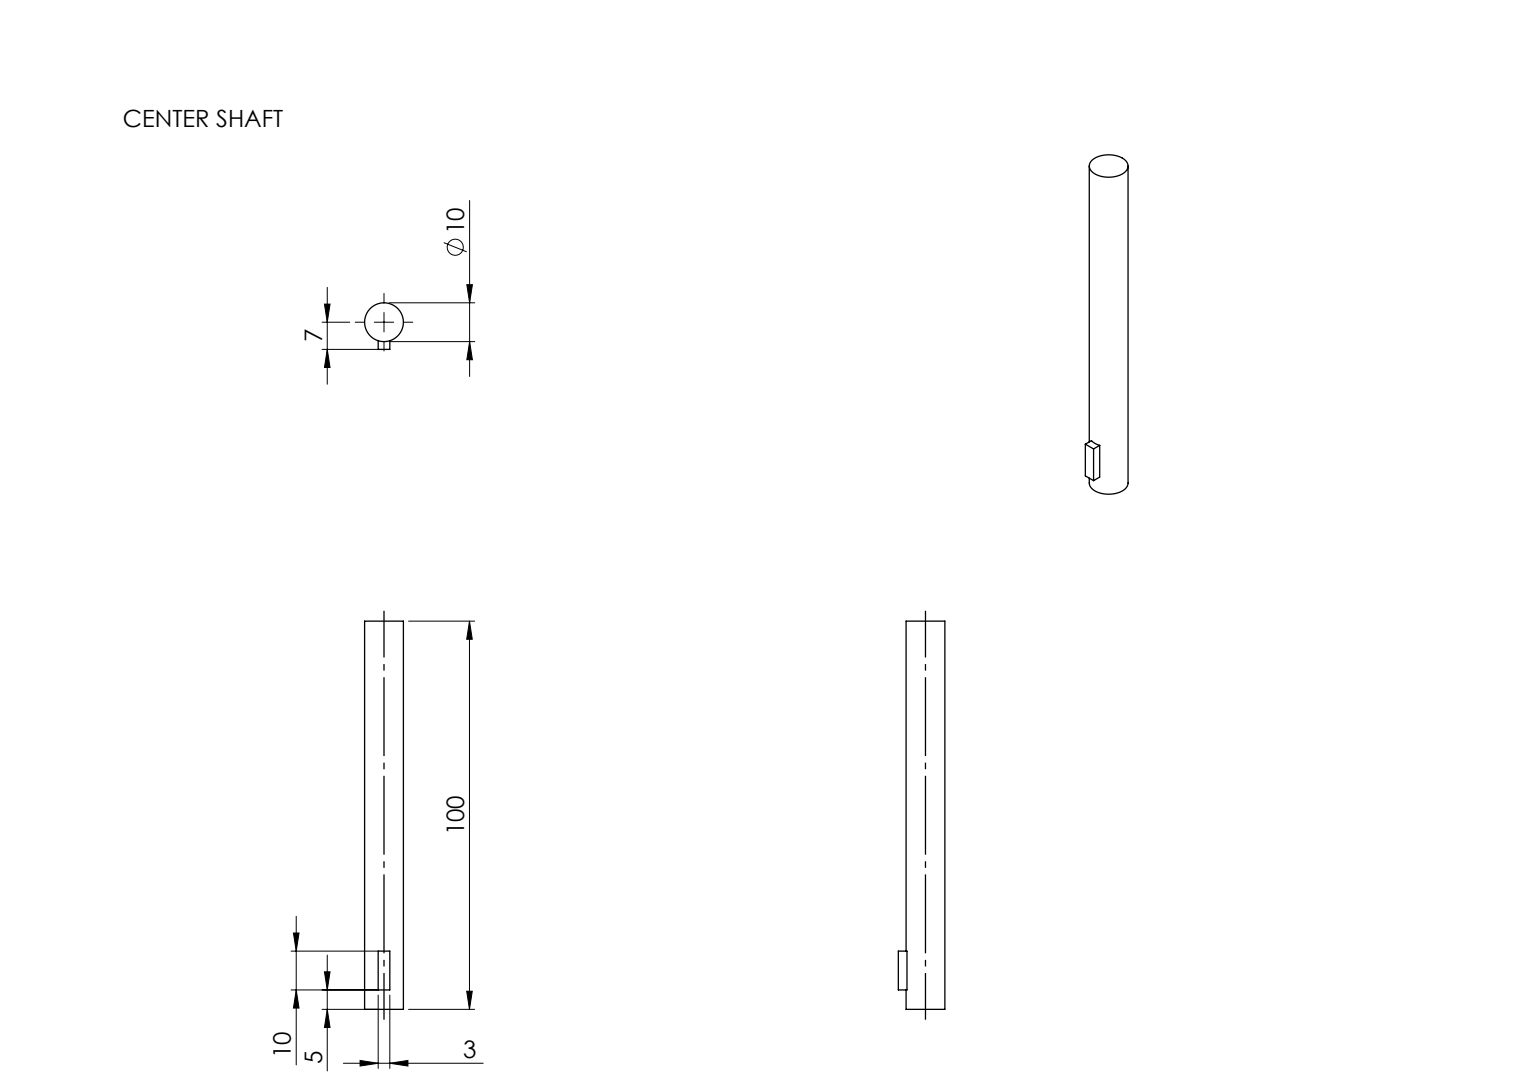
ISO-10303-21;
HEADER;
FILE_DESCRIPTION (('STEP AP214'),
    '1' );
FILE_NAME ('center shaft.step',
    '2026-09-30T13:58:28',
    ( '' ),
    ( '' ),
    'SwSTEP 2.0',
    'SolidWorks 2026',
    '' );
FILE_SCHEMA (( 'AUTOMOTIVE_DESIGN' ));
ENDSEC;

DATA;
#92=CARTESIAN_POINT ( 'NONE',  ( 0.000000000000000000, 100.0000000000000000, 0.000000000000000000 ) ) ;
#95=ADVANCED_FACE ( 'NONE', ( #16404 ), #1281, .F. ) ;
#101=PRODUCT_DEFINITION ( 'UNKNOWN', '', #429, #16859 ) ;
#199=CLOSED_SHELL ( 'NONE', ( #12068, #15575, #17594, #6767, #11084, #7759, #19088, #8385, #95 ) ) ;
#265=EDGE_LOOP ( 'NONE', ( #20128, #1055, #4125, #2694 ) ) ;
#321=EDGE_CURVE ( 'NONE', #616, #3222, #16347, .T. ) ;
#429=PRODUCT_DEFINITION_FORMATION_WITH_SPECIFIED_SOURCE ( 'ANY', '', #11974, .NOT_KNOWN. ) ;
#455=AXIS2_PLACEMENT_3D ( 'NONE', #21743, #16562, #6840 ) ;
#607=DIRECTION ( 'NONE',  ( 0.000000000000000000, 0.000000000000000000, 1.000000000000000000 ) ) ;
#616=VERTEX_POINT ( 'NONE', #12037 ) ;
#674=CARTESIAN_POINT ( 'NONE',  ( 0.000000000000000000, 100.0000000000000000, 0.000000000000000000 ) ) ;
#683=MECHANICAL_DESIGN_GEOMETRIC_PRESENTATION_REPRESENTATION('',(#2802),#19738);
#725=( NAMED_UNIT ( * ) PLANE_ANGLE_UNIT ( ) SI_UNIT ( $, .RADIAN. ) );
#742=EDGE_CURVE ( 'NONE', #12477, #5806, #14229, .T. ) ;
#798=LINE ( 'NONE', #17288, #11093 ) ;
#800=VECTOR ( 'NONE', #14018, 1000.000000000000000 ) ;
#823=FILL_AREA_STYLE_COLOUR ( '', #19105 ) ;
#989=ORIENTED_EDGE ( 'NONE', *, *, #9839, .T. ) ;
#1055=ORIENTED_EDGE ( 'NONE', *, *, #8824, .T. ) ;
#1127=VERTEX_POINT ( 'NONE', #4265 ) ;
#1209=VECTOR ( 'NONE', #5021, 1000.000000000000000 ) ;
#1226=CARTESIAN_POINT ( 'NONE',  ( -1.500000000000000000, 5.000000000000000000, 7.000000000000000000 ) ) ;
#1281=PLANE ( 'NONE',  #4780 ) ;
#1293=DIRECTION ( 'NONE',  ( 0.000000000000000000, -1.000000000000000000, 0.000000000000000000 ) ) ;
#1344=AXIS2_PLACEMENT_3D ( 'NONE', #6692, #13295, #13408 ) ;
#1351=CARTESIAN_POINT ( 'NONE',  ( -1.500000000000000000, 15.00000000000000000, 7.000000000000000000 ) ) ;
#1432=PLANE ( 'NONE',  #13990 ) ;
#1507=ORIENTED_EDGE ( 'NONE', *, *, #15912, .F. ) ;
#1509=ORIENTED_EDGE ( 'NONE', *, *, #20060, .F. ) ;
#1631=APPLICATION_CONTEXT ( 'automotive_design' ) ;
#1753=FACE_OUTER_BOUND ( 'NONE', #3852, .T. ) ;
#1932=ORIENTED_EDGE ( 'NONE', *, *, #19995, .T. ) ;
#1943=( NAMED_UNIT ( * ) PLANE_ANGLE_UNIT ( ) SI_UNIT ( $, .RADIAN. ) );
#2032=DIRECTION ( 'NONE',  ( 0.000000000000000000, 0.000000000000000000, 1.000000000000000000 ) ) ;
#2075=CIRCLE ( 'NONE', #19698, 5.000000000000000000 ) ;
#2102=CARTESIAN_POINT ( 'NONE',  ( 0.000000000000000000, 100.0000000000000000, -5.000000000000000000 ) ) ;
#2151=LINE ( 'NONE', #5477, #19260 ) ;
#2243=DIRECTION ( 'NONE',  ( 0.000000000000000000, 0.000000000000000000, 1.000000000000000000 ) ) ;
#2374=SURFACE_STYLE_USAGE ( .BOTH. , #7253 ) ;
#2502=FACE_OUTER_BOUND ( 'NONE', #20642, .T. ) ;
#2509=ORIENTED_EDGE ( 'NONE', *, *, #11386, .F. ) ;
#2694=ORIENTED_EDGE ( 'NONE', *, *, #321, .F. ) ;
#2772=CARTESIAN_POINT ( 'NONE',  ( -1.500000000000000000, 15.00000000000000000, 0.000000000000000000 ) ) ;
#2791=EDGE_LOOP ( 'NONE', ( #1507, #989, #4089, #3085, #18940 ) ) ;
#2802=STYLED_ITEM ( 'NONE', ( #15197 ), #20649 ) ;
#2947=LINE ( 'NONE', #9672, #7434 ) ;
#2951=CYLINDRICAL_SURFACE ( 'NONE', #10092, 5.000000000000000000 ) ;
#3085=ORIENTED_EDGE ( 'NONE', *, *, #321, .T. ) ;
#3145=FACE_OUTER_BOUND ( 'NONE', #265, .T. ) ;
#3179=CARTESIAN_POINT ( 'NONE',  ( 0.000000000000000000, 100.0000000000000000, 0.000000000000000000 ) ) ;
#3220=PRODUCT_CONTEXT ( 'NONE', #1631, 'mechanical' ) ;
#3222=VERTEX_POINT ( 'NONE', #17271 ) ;
#3230=CARTESIAN_POINT ( 'NONE',  ( 0.000000000000000000, 100.0000000000000000, -5.000000000000000000 ) ) ;
#3247=PLANE ( 'NONE',  #11760 ) ;
#3300=VERTEX_POINT ( 'NONE', #14049 ) ;
#3320=PRODUCT_DEFINITION_SHAPE ( 'NONE', 'NONE',  #101 ) ;
#3361=CARTESIAN_POINT ( 'NONE',  ( 0.000000000000000000, 5.000000000000004441, 0.000000000000000000 ) ) ;
#3443=ORIENTED_EDGE ( 'NONE', *, *, #17842, .T. ) ;
#3468=ORIENTED_EDGE ( 'NONE', *, *, #18425, .F. ) ;
#3530=VERTEX_POINT ( 'NONE', #1226 ) ;
#3670=EDGE_LOOP ( 'NONE', ( #9750, #16754, #6405, #15038, #9979 ) ) ;
#3852=EDGE_LOOP ( 'NONE', ( #3468, #5746 ) ) ;
#3925=( GEOMETRIC_REPRESENTATION_CONTEXT ( 3 ) GLOBAL_UNCERTAINTY_ASSIGNED_CONTEXT ( ( #11439 ) ) GLOBAL_UNIT_ASSIGNED_CONTEXT ( ( #13771, #12002, #13329 ) ) REPRESENTATION_CONTEXT ( 'NONE', 'WORKASPACE' ) );
#4089=ORIENTED_EDGE ( 'NONE', *, *, #13808, .T. ) ;
#4125=ORIENTED_EDGE ( 'NONE', *, *, #12182, .F. ) ;
#4147=( NAMED_UNIT ( * ) SI_UNIT ( $, .STERADIAN. ) SOLID_ANGLE_UNIT ( ) );
#4205=ORIENTED_EDGE ( 'NONE', *, *, #742, .T. ) ;
#4244=CARTESIAN_POINT ( 'NONE',  ( 6.123233995736766282E-16, 100.0000000000000000, 5.000000000000000000 ) ) ;
#4265=CARTESIAN_POINT ( 'NONE',  ( 6.123233995736766282E-16, 0.000000000000000000, 5.000000000000000000 ) ) ;
#4349=EDGE_CURVE ( 'NONE', #20466, #11655, #2075, .T. ) ;
#4384=CARTESIAN_POINT ( 'NONE',  ( -1.500000000000000000, 5.000000000000000000, 7.000000000000000000 ) ) ;
#4780=AXIS2_PLACEMENT_3D ( 'NONE', #19941, #11549, #8018 ) ;
#4823=DIRECTION ( 'NONE',  ( 0.000000000000000000, 0.000000000000000000, -1.000000000000000000 ) ) ;
#4851=VECTOR ( 'NONE', #14439, 1000.000000000000000 ) ;
#4937=COLOUR_RGB ( '', 0.09019608, 0.27058824, 0.51372549) ;
#5017=DIRECTION ( 'NONE',  ( -0.000000000000000000, 0.000000000000000000, -1.000000000000000000 ) ) ;
#5021=DIRECTION ( 'NONE',  ( 0.000000000000000000, -1.000000000000000000, 0.000000000000000000 ) ) ;
#5043=SURFACE_STYLE_USAGE ( .BOTH. , #13323 ) ;
#5212=LINE ( 'NONE', #10500, #21204 ) ;
#5238=CARTESIAN_POINT ( 'NONE',  ( -1.500000000000000000, 5.000000000000004441, 4.769696007084728073 ) ) ;
#5247=LINE ( 'NONE', #15394, #1209 ) ;
#5477=CARTESIAN_POINT ( 'NONE',  ( 1.500000000000000000, 15.00000000000000000, 0.000000000000000000 ) ) ;
#5531=DIRECTION ( 'NONE',  ( 0.000000000000000000, 0.000000000000000000, 1.000000000000000000 ) ) ;
#5556=CARTESIAN_POINT ( 'NONE',  ( 6.123233995736766282E-16, 15.00000000000000000, 5.000000000000000000 ) ) ;
#5679=( GEOMETRIC_REPRESENTATION_CONTEXT ( 3 ) GLOBAL_UNCERTAINTY_ASSIGNED_CONTEXT ( ( #16530 ) ) GLOBAL_UNIT_ASSIGNED_CONTEXT ( ( #15634, #725, #4147 ) ) REPRESENTATION_CONTEXT ( 'NONE', 'WORKASPACE' ) );
#5746=ORIENTED_EDGE ( 'NONE', *, *, #4349, .F. ) ;
#5806=VERTEX_POINT ( 'NONE', #10160 ) ;
#5839=FACE_OUTER_BOUND ( 'NONE', #21460, .T. ) ;
#5917=SHAPE_REPRESENTATION_RELATIONSHIP ( 'NONE' , 'NONE' ,  #21798, #14875 ) ;
#5959=VECTOR ( 'NONE', #11292, 1000.000000000000000 ) ;
#6120=VECTOR ( 'NONE', #9359, 1000.000000000000000 ) ;
#6326=EDGE_CURVE ( 'NONE', #9874, #3300, #9010, .T. ) ;
#6373=EDGE_LOOP ( 'NONE', ( #19171, #4205, #13352, #17793 ) ) ;
#6384=CARTESIAN_POINT ( 'NONE',  ( 1.500000000000000000, 15.00000000000000000, 0.000000000000000000 ) ) ;
#6386=UNCERTAINTY_MEASURE_WITH_UNIT (LENGTH_MEASURE( 1.000000000000000082E-05 ), #11681, 'distance_accuracy_value', 'NONE');
#6403=DIRECTION ( 'NONE',  ( 0.000000000000000000, -1.000000000000000000, 0.000000000000000000 ) ) ;
#6405=ORIENTED_EDGE ( 'NONE', *, *, #17842, .F. ) ;
#6414=STYLED_ITEM ( 'NONE', ( #19070 ), #14875 ) ;
#6551=ORIENTED_EDGE ( 'NONE', *, *, #21621, .T. ) ;
#6596=PLANE ( 'NONE',  #17058 ) ;
#6692=CARTESIAN_POINT ( 'NONE',  ( 0.000000000000000000, 100.0000000000000000, 0.000000000000000000 ) ) ;
#6767=ADVANCED_FACE ( 'NONE', ( #12202 ), #6917, .T. ) ;
#6840=DIRECTION ( 'NONE',  ( 0.000000000000000000, 0.000000000000000000, 1.000000000000000000 ) ) ;
#6917=PLANE ( 'NONE',  #14621 ) ;
#6948=CARTESIAN_POINT ( 'NONE',  ( 1.500000000000000000, 15.00000000000000000, 7.000000000000000000 ) ) ;
#7066=ORIENTED_EDGE ( 'NONE', *, *, #7566, .T. ) ;
#7140=FACE_OUTER_BOUND ( 'NONE', #2791, .T. ) ;
#7253=SURFACE_SIDE_STYLE ('',( #20728 ) ) ;
#7366=FILL_AREA_STYLE ('',( #823 ) ) ;
#7418=DIRECTION ( 'NONE',  ( 0.000000000000000000, -1.000000000000000000, 0.000000000000000000 ) ) ;
#7419=ORIENTED_EDGE ( 'NONE', *, *, #8672, .T. ) ;
#7434=VECTOR ( 'NONE', #18325, 1000.000000000000000 ) ;
#7467=ORIENTED_EDGE ( 'NONE', *, *, #11386, .T. ) ;
#7566=EDGE_CURVE ( 'NONE', #11073, #19781, #13486, .T. ) ;
#7614=DIRECTION ( 'NONE',  ( -0.000000000000000000, -1.000000000000000000, -0.000000000000000000 ) ) ;
#7759=ADVANCED_FACE ( 'NONE', ( #3145 ), #3247, .F. ) ;
#8018=DIRECTION ( 'NONE',  ( -1.000000000000000000, 0.000000000000000000, 0.000000000000000000 ) ) ;
#8056=CIRCLE ( 'NONE', #1344, 5.000000000000000000 ) ;
#8276=DIRECTION ( 'NONE',  ( 0.000000000000000000, -1.000000000000000000, 0.000000000000000000 ) ) ;
#8358=( NAMED_UNIT ( * ) SI_UNIT ( $, .STERADIAN. ) SOLID_ANGLE_UNIT ( ) );
#8385=ADVANCED_FACE ( 'NONE', ( #7140 ), #17414, .T. ) ;
#8462=DIRECTION ( 'NONE',  ( 0.000000000000000000, -0.000000000000000000, -1.000000000000000000 ) ) ;
#8616=CIRCLE ( 'NONE', #15680, 5.000000000000000000 ) ;
#8628=EDGE_CURVE ( 'NONE', #12477, #11073, #19544, .T. ) ;
#8670=CARTESIAN_POINT ( 'NONE',  ( 0.000000000000000000, 0.000000000000000000, 0.000000000000000000 ) ) ;
#8672=EDGE_CURVE ( 'NONE', #11073, #1127, #5247, .T. ) ;
#8824=EDGE_CURVE ( 'NONE', #19781, #3530, #798, .T. ) ;
#9010=LINE ( 'NONE', #6948, #18478 ) ;
#9228=CYLINDRICAL_SURFACE ( 'NONE', #11282, 5.000000000000000000 ) ;
#9258=ORIENTED_EDGE ( 'NONE', *, *, #8628, .T. ) ;
#9359=DIRECTION ( 'NONE',  ( -0.000000000000000000, 1.000000000000000000, -0.000000000000000000 ) ) ;
#9456=PLANE ( 'NONE',  #12316 ) ;
#9564=CARTESIAN_POINT ( 'NONE',  ( -1.500000000000000000, 15.00000000000000000, 7.000000000000000000 ) ) ;
#9591=ORIENTED_EDGE ( 'NONE', *, *, #4349, .T. ) ;
#9672=CARTESIAN_POINT ( 'NONE',  ( -1.500000000000000000, 100.0000000000000000, 4.769696007084728073 ) ) ;
#9750=ORIENTED_EDGE ( 'NONE', *, *, #8628, .F. ) ;
#9839=EDGE_CURVE ( 'NONE', #5806, #18737, #8616, .T. ) ;
#9874=VERTEX_POINT ( 'NONE', #14862 ) ;
#9921=CARTESIAN_POINT ( 'NONE',  ( 0.000000000000000000, 0.000000000000000000, 0.000000000000000000 ) ) ;
#9977=DIRECTION ( 'NONE',  ( 1.000000000000000000, 0.000000000000000000, -0.000000000000000000 ) ) ;
#9979=ORIENTED_EDGE ( 'NONE', *, *, #7566, .F. ) ;
#10092=AXIS2_PLACEMENT_3D ( 'NONE', #3179, #6403, #16434 ) ;
#10097=DIRECTION ( 'NONE',  ( -3.552713678800500929E-15, 0.000000000000000000, 1.000000000000000000 ) ) ;
#10160=CARTESIAN_POINT ( 'NONE',  ( 1.500000000000000000, 15.00000000000000000, 4.769696007084728073 ) ) ;
#10500=CARTESIAN_POINT ( 'NONE',  ( 1.500000000000000000, 5.000000000000000000, 0.000000000000000000 ) ) ;
#10564=DIRECTION ( 'NONE',  ( -1.000000000000000000, 0.000000000000000000, 0.000000000000000000 ) ) ;
#10567=ORIENTED_EDGE ( 'NONE', *, *, #13808, .F. ) ;
#10583=ORIENTED_EDGE ( 'NONE', *, *, #10930, .T. ) ;
#10598=LINE ( 'NONE', #2102, #800 ) ;
#10728=AXIS2_PLACEMENT_3D ( 'NONE', #3361, #15069, #10097 ) ;
#10930=EDGE_CURVE ( 'NONE', #11655, #11594, #10598, .T. ) ;
#11023=DIRECTION ( 'NONE',  ( 1.000000000000000000, 0.000000000000000000, -0.000000000000000000 ) ) ;
#11073=VERTEX_POINT ( 'NONE', #15997 ) ;
#11084=ADVANCED_FACE ( 'NONE', ( #13196 ), #6596, .T. ) ;
#11093=VECTOR ( 'NONE', #2032, 1000.000000000000000 ) ;
#11239=DIRECTION ( 'NONE',  ( -1.000000000000000000, 0.000000000000000000, -0.000000000000000000 ) ) ;
#11254=AXIS2_PLACEMENT_3D ( 'NONE', #9921, #16663, #12789 ) ;
#11282=AXIS2_PLACEMENT_3D ( 'NONE', #18312, #1293, #4823 ) ;
#11292=DIRECTION ( 'NONE',  ( 1.000000000000000000, 0.000000000000000000, 0.000000000000000000 ) ) ;
#11386=EDGE_CURVE ( 'NONE', #20466, #18737, #17396, .T. ) ;
#11439=UNCERTAINTY_MEASURE_WITH_UNIT (LENGTH_MEASURE( 1.000000000000000082E-05 ), #13771, 'distance_accuracy_value', 'NONE');
#11537=AXIS2_PLACEMENT_3D ( 'NONE', #17455, #7614, #19323 ) ;
#11549=DIRECTION ( 'NONE',  ( 0.000000000000000000, 1.000000000000000000, 0.000000000000000000 ) ) ;
#11594=VERTEX_POINT ( 'NONE', #16499 ) ;
#11655=VERTEX_POINT ( 'NONE', #3230 ) ;
#11681=( LENGTH_UNIT ( ) NAMED_UNIT ( * ) SI_UNIT ( .MILLI., .METRE. ) );
#11760=AXIS2_PLACEMENT_3D ( 'NONE', #13301, #9977, #5017 ) ;
#11974=PRODUCT ( 'center shaft', 'center shaft', '', ( #3220 ) ) ;
#12002=( NAMED_UNIT ( * ) PLANE_ANGLE_UNIT ( ) SI_UNIT ( $, .RADIAN. ) );
#12037=CARTESIAN_POINT ( 'NONE',  ( -1.500000000000000000, 15.00000000000000000, 4.769696007084728073 ) ) ;
#12068=ADVANCED_FACE ( 'NONE', ( #17999 ), #2951, .T. ) ;
#12133=AXIS2_PLACEMENT_3D ( 'NONE', #12540, #20617, #10564 ) ;
#12182=EDGE_CURVE ( 'NONE', #3222, #3530, #21295, .T. ) ;
#12202=FACE_OUTER_BOUND ( 'NONE', #16612, .T. ) ;
#12316=AXIS2_PLACEMENT_3D ( 'NONE', #17764, #19307, #11239 ) ;
#12375=ORIENTED_EDGE ( 'NONE', *, *, #12182, .T. ) ;
#12423=VECTOR ( 'NONE', #2243, 1000.000000000000000 ) ;
#12477=VERTEX_POINT ( 'NONE', #20950 ) ;
#12500=DIRECTION ( 'NONE',  ( 0.000000000000000000, 0.000000000000000000, -1.000000000000000000 ) ) ;
#12540=CARTESIAN_POINT ( 'NONE',  ( 0.000000000000000000, 15.00000000000000000, 0.000000000000000000 ) ) ;
#12662=CIRCLE ( 'NONE', #11254, 5.000000000000000000 ) ;
#12789=DIRECTION ( 'NONE',  ( 0.000000000000000000, 0.000000000000000000, -1.000000000000000000 ) ) ;
#12997=CIRCLE ( 'NONE', #21816, 5.000000000000000000 ) ;
#13196=FACE_OUTER_BOUND ( 'NONE', #6373, .T. ) ;
#13295=DIRECTION ( 'NONE',  ( 0.000000000000000000, -1.000000000000000000, 0.000000000000000000 ) ) ;
#13301=CARTESIAN_POINT ( 'NONE',  ( -1.500000000000000000, 15.00000000000000000, 0.000000000000000000 ) ) ;
#13323=SURFACE_SIDE_STYLE ('',( #17081 ) ) ;
#13329=( NAMED_UNIT ( * ) SI_UNIT ( $, .STERADIAN. ) SOLID_ANGLE_UNIT ( ) );
#13352=ORIENTED_EDGE ( 'NONE', *, *, #15912, .T. ) ;
#13408=DIRECTION ( 'NONE',  ( 0.000000000000000000, 0.000000000000000000, -1.000000000000000000 ) ) ;
#13486=CIRCLE ( 'NONE', #455, 5.000000000000000000 ) ;
#13771=( LENGTH_UNIT ( ) NAMED_UNIT ( * ) SI_UNIT ( .MILLI., .METRE. ) );
#13808=EDGE_CURVE ( 'NONE', #18737, #616, #16831, .T. ) ;
#13990=AXIS2_PLACEMENT_3D ( 'NONE', #92, #8276, #16667 ) ;
#14018=DIRECTION ( 'NONE',  ( 0.000000000000000000, -1.000000000000000000, 0.000000000000000000 ) ) ;
#14049=CARTESIAN_POINT ( 'NONE',  ( 1.500000000000000000, 5.000000000000000000, 7.000000000000000000 ) ) ;
#14229=LINE ( 'NONE', #15993, #6120 ) ;
#14439=DIRECTION ( 'NONE',  ( 1.000000000000000000, 0.000000000000000000, 0.000000000000000000 ) ) ;
#14533=CARTESIAN_POINT ( 'NONE',  ( 0.000000000000000000, 15.00000000000000000, 0.000000000000000000 ) ) ;
#14553=DIRECTION ( 'NONE',  ( 0.000000000000000000, -1.000000000000000000, 0.000000000000000000 ) ) ;
#14621=AXIS2_PLACEMENT_3D ( 'NONE', #8670, #18839, #8462 ) ;
#14776=ORIENTED_EDGE ( 'NONE', *, *, #15183, .T. ) ;
#14862=CARTESIAN_POINT ( 'NONE',  ( 1.500000000000000000, 15.00000000000000000, 7.000000000000000000 ) ) ;
#14875=ADVANCED_BREP_SHAPE_REPRESENTATION ( '', ( #20649, #15567 ), #3925 ) ;
#14971=ORIENTED_EDGE ( 'NONE', *, *, #742, .F. ) ;
#15038=ORIENTED_EDGE ( 'NONE', *, *, #8824, .F. ) ;
#15045=SHAPE_DEFINITION_REPRESENTATION ( #3320, #21798 ) ;
#15069=DIRECTION ( 'NONE',  ( -0.000000000000000000, -1.000000000000000000, -0.000000000000000000 ) ) ;
#15183=EDGE_CURVE ( 'NONE', #1127, #11594, #12662, .T. ) ;
#15197=PRESENTATION_STYLE_ASSIGNMENT (( #5043 ) ) ;
#15394=CARTESIAN_POINT ( 'NONE',  ( 6.123233995736766282E-16, 100.0000000000000000, 5.000000000000000000 ) ) ;
#15434=DIRECTION ( 'NONE',  ( 0.000000000000000000, -1.000000000000000000, 0.000000000000000000 ) ) ;
#15567=AXIS2_PLACEMENT_3D ( 'NONE', #21837, #20187, #17085 ) ;
#15575=ADVANCED_FACE ( 'NONE', ( #2502 ), #9228, .T. ) ;
#15634=( LENGTH_UNIT ( ) NAMED_UNIT ( * ) SI_UNIT ( .MILLI., .METRE. ) );
#15680=AXIS2_PLACEMENT_3D ( 'NONE', #14533, #19944, #21275 ) ;
#15886=CARTESIAN_POINT ( 'NONE',  ( 6.123233995736766282E-16, 100.0000000000000000, 5.000000000000000000 ) ) ;
#15912=EDGE_CURVE ( 'NONE', #5806, #9874, #2151, .T. ) ;
#15993=CARTESIAN_POINT ( 'NONE',  ( 1.500000000000000000, 100.0000000000000000, 4.769696007084728073 ) ) ;
#15997=CARTESIAN_POINT ( 'NONE',  ( 6.123233995736766282E-16, 5.000000000000004441, 5.000000000000000000 ) ) ;
#16347=LINE ( 'NONE', #2772, #12423 ) ;
#16404=FACE_OUTER_BOUND ( 'NONE', #3670, .T. ) ;
#16434=DIRECTION ( 'NONE',  ( 0.000000000000000000, 0.000000000000000000, -1.000000000000000000 ) ) ;
#16499=CARTESIAN_POINT ( 'NONE',  ( 0.000000000000000000, 0.000000000000000000, -5.000000000000000000 ) ) ;
#16530=UNCERTAINTY_MEASURE_WITH_UNIT (LENGTH_MEASURE( 1.000000000000000082E-05 ), #15634, 'distance_accuracy_value', 'NONE');
#16562=DIRECTION ( 'NONE',  ( -0.000000000000000000, -1.000000000000000000, -0.000000000000000000 ) ) ;
#16572=ORIENTED_EDGE ( 'NONE', *, *, #8672, .F. ) ;
#16612=EDGE_LOOP ( 'NONE', ( #1932, #14776 ) ) ;
#16636=DIRECTION ( 'NONE',  ( -0.000000000000000000, 0.000000000000000000, -1.000000000000000000 ) ) ;
#16663=DIRECTION ( 'NONE',  ( 0.000000000000000000, -1.000000000000000000, 0.000000000000000000 ) ) ;
#16667=DIRECTION ( 'NONE',  ( 0.000000000000000000, -0.000000000000000000, -1.000000000000000000 ) ) ;
#16673=ORIENTED_EDGE ( 'NONE', *, *, #10930, .F. ) ;
#16754=ORIENTED_EDGE ( 'NONE', *, *, #21484, .T. ) ;
#16831=CIRCLE ( 'NONE', #11537, 5.000000000000000000 ) ;
#16859=PRODUCT_DEFINITION_CONTEXT ( 'detailed design', #19692, 'design' ) ;
#16956=ORIENTED_EDGE ( 'NONE', *, *, #19995, .F. ) ;
#17032=DIRECTION ( 'NONE',  ( 0.000000000000000000, 0.000000000000000000, -1.000000000000000000 ) ) ;
#17058=AXIS2_PLACEMENT_3D ( 'NONE', #6384, #11023, #16636 ) ;
#17081=SURFACE_STYLE_FILL_AREA ( #20080 ) ;
#17085=DIRECTION ( 'NONE',  ( 1.000000000000000000, 0.000000000000000000, 0.000000000000000000 ) ) ;
#17271=CARTESIAN_POINT ( 'NONE',  ( -1.500000000000000000, 15.00000000000000000, 7.000000000000000000 ) ) ;
#17288=CARTESIAN_POINT ( 'NONE',  ( -1.500000000000000000, 5.000000000000000000, 0.000000000000000000 ) ) ;
#17396=LINE ( 'NONE', #4244, #21310 ) ;
#17414=PLANE ( 'NONE',  #12133 ) ;
#17455=CARTESIAN_POINT ( 'NONE',  ( 0.000000000000000000, 15.00000000000000000, 0.000000000000000000 ) ) ;
#17594=ADVANCED_FACE ( 'NONE', ( #1753 ), #1432, .F. ) ;
#17684=MECHANICAL_DESIGN_GEOMETRIC_PRESENTATION_REPRESENTATION('',(#6414),#5679);
#17742=ORIENTED_EDGE ( 'NONE', *, *, #18425, .T. ) ;
#17764=CARTESIAN_POINT ( 'NONE',  ( -1.500000000000000000, 15.00000000000000000, 7.000000000000000000 ) ) ;
#17793=ORIENTED_EDGE ( 'NONE', *, *, #6326, .T. ) ;
#17833=DIRECTION ( 'NONE',  ( 0.000000000000000000, -1.000000000000000000, 0.000000000000000000 ) ) ;
#17842=EDGE_CURVE ( 'NONE', #3530, #3300, #17875, .T. ) ;
#17875=LINE ( 'NONE', #4384, #4851 ) ;
#17999=FACE_OUTER_BOUND ( 'NONE', #18572, .T. ) ;
#18233=ORIENTED_EDGE ( 'NONE', *, *, #6326, .F. ) ;
#18312=CARTESIAN_POINT ( 'NONE',  ( 0.000000000000000000, 100.0000000000000000, 0.000000000000000000 ) ) ;
#18325=DIRECTION ( 'NONE',  ( -0.000000000000000000, 1.000000000000000000, -0.000000000000000000 ) ) ;
#18425=EDGE_CURVE ( 'NONE', #11655, #20466, #8056, .T. ) ;
#18478=VECTOR ( 'NONE', #15434, 1000.000000000000000 ) ;
#18531=VECTOR ( 'NONE', #14553, 1000.000000000000000 ) ;
#18572=EDGE_LOOP ( 'NONE', ( #17742, #7467, #19840, #14971, #9258, #7419, #16956, #16673 ) ) ;
#18737=VERTEX_POINT ( 'NONE', #5556 ) ;
#18839=DIRECTION ( 'NONE',  ( 0.000000000000000000, -1.000000000000000000, 0.000000000000000000 ) ) ;
#18940=ORIENTED_EDGE ( 'NONE', *, *, #20060, .T. ) ;
#19070=PRESENTATION_STYLE_ASSIGNMENT (( #2374 ) ) ;
#19088=ADVANCED_FACE ( 'NONE', ( #5839 ), #9456, .F. ) ;
#19105=COLOUR_RGB ( '', 0.09019608, 0.27058824, 0.51372549) ;
#19171=ORIENTED_EDGE ( 'NONE', *, *, #21484, .F. ) ;
#19260=VECTOR ( 'NONE', #607, 1000.000000000000000 ) ;
#19307=DIRECTION ( 'NONE',  ( 0.000000000000000000, 0.000000000000000000, -1.000000000000000000 ) ) ;
#19323=DIRECTION ( 'NONE',  ( 0.000000000000000000, 0.000000000000000000, 1.000000000000000000 ) ) ;
#19465=CARTESIAN_POINT ( 'NONE',  ( 0.000000000000000000, 0.000000000000000000, 0.000000000000000000 ) ) ;
#19544=CIRCLE ( 'NONE', #10728, 5.000000000000000000 ) ;
#19692=APPLICATION_CONTEXT ( 'automotive_design' ) ;
#19698=AXIS2_PLACEMENT_3D ( 'NONE', #674, #7418, #17032 ) ;
#19738=( GEOMETRIC_REPRESENTATION_CONTEXT ( 3 ) GLOBAL_UNCERTAINTY_ASSIGNED_CONTEXT ( ( #6386 ) ) GLOBAL_UNIT_ASSIGNED_CONTEXT ( ( #11681, #1943, #8358 ) ) REPRESENTATION_CONTEXT ( 'NONE', 'WORKASPACE' ) );
#19781=VERTEX_POINT ( 'NONE', #5238 ) ;
#19799=LINE ( 'NONE', #1351, #5959 ) ;
#19840=ORIENTED_EDGE ( 'NONE', *, *, #9839, .F. ) ;
#19941=CARTESIAN_POINT ( 'NONE',  ( 0.000000000000000000, 5.000000000000000000, 0.000000000000000000 ) ) ;
#19944=DIRECTION ( 'NONE',  ( -0.000000000000000000, -1.000000000000000000, -0.000000000000000000 ) ) ;
#19995=EDGE_CURVE ( 'NONE', #11594, #1127, #12997, .T. ) ;
#20060=EDGE_CURVE ( 'NONE', #3222, #9874, #19799, .T. ) ;
#20080=FILL_AREA_STYLE ('',( #21724 ) ) ;
#20128=ORIENTED_EDGE ( 'NONE', *, *, #21621, .F. ) ;
#20187=DIRECTION ( 'NONE',  ( 0.000000000000000000, 0.000000000000000000, 1.000000000000000000 ) ) ;
#20466=VERTEX_POINT ( 'NONE', #15886 ) ;
#20556=ORIENTED_EDGE ( 'NONE', *, *, #15183, .F. ) ;
#20617=DIRECTION ( 'NONE',  ( 0.000000000000000000, 1.000000000000000000, 0.000000000000000000 ) ) ;
#20642=EDGE_LOOP ( 'NONE', ( #2509, #9591, #10583, #20556, #16572, #7066, #6551, #10567 ) ) ;
#20649=MANIFOLD_SOLID_BREP ( 'Extrude-Thin1', #199 ) ;
#20728=SURFACE_STYLE_FILL_AREA ( #7366 ) ;
#20905=DIRECTION ( 'NONE',  ( 0.000000000000000000, -1.000000000000000000, 0.000000000000000000 ) ) ;
#20950=CARTESIAN_POINT ( 'NONE',  ( 1.500000000000000000, 5.000000000000004441, 4.769696007084728073 ) ) ;
#21204=VECTOR ( 'NONE', #5531, 1000.000000000000000 ) ;
#21275=DIRECTION ( 'NONE',  ( -3.552713678800500929E-15, 0.000000000000000000, 1.000000000000000000 ) ) ;
#21295=LINE ( 'NONE', #9564, #18531 ) ;
#21310=VECTOR ( 'NONE', #17833, 1000.000000000000000 ) ;
#21460=EDGE_LOOP ( 'NONE', ( #3443, #18233, #1509, #12375 ) ) ;
#21484=EDGE_CURVE ( 'NONE', #12477, #3300, #5212, .T. ) ;
#21621=EDGE_CURVE ( 'NONE', #19781, #616, #2947, .T. ) ;
#21724=FILL_AREA_STYLE_COLOUR ( '', #4937 ) ;
#21743=CARTESIAN_POINT ( 'NONE',  ( 0.000000000000000000, 5.000000000000004441, 0.000000000000000000 ) ) ;
#21798=SHAPE_REPRESENTATION ( 'center shaft', ( #15567 ), #3925 ) ;
#21816=AXIS2_PLACEMENT_3D ( 'NONE', #19465, #20905, #12500 ) ;
#21837=CARTESIAN_POINT ( 'NONE',  ( 0.000000000000000000, 0.000000000000000000, 0.000000000000000000 ) ) ;
ENDSEC;
END-ISO-10303-21;
